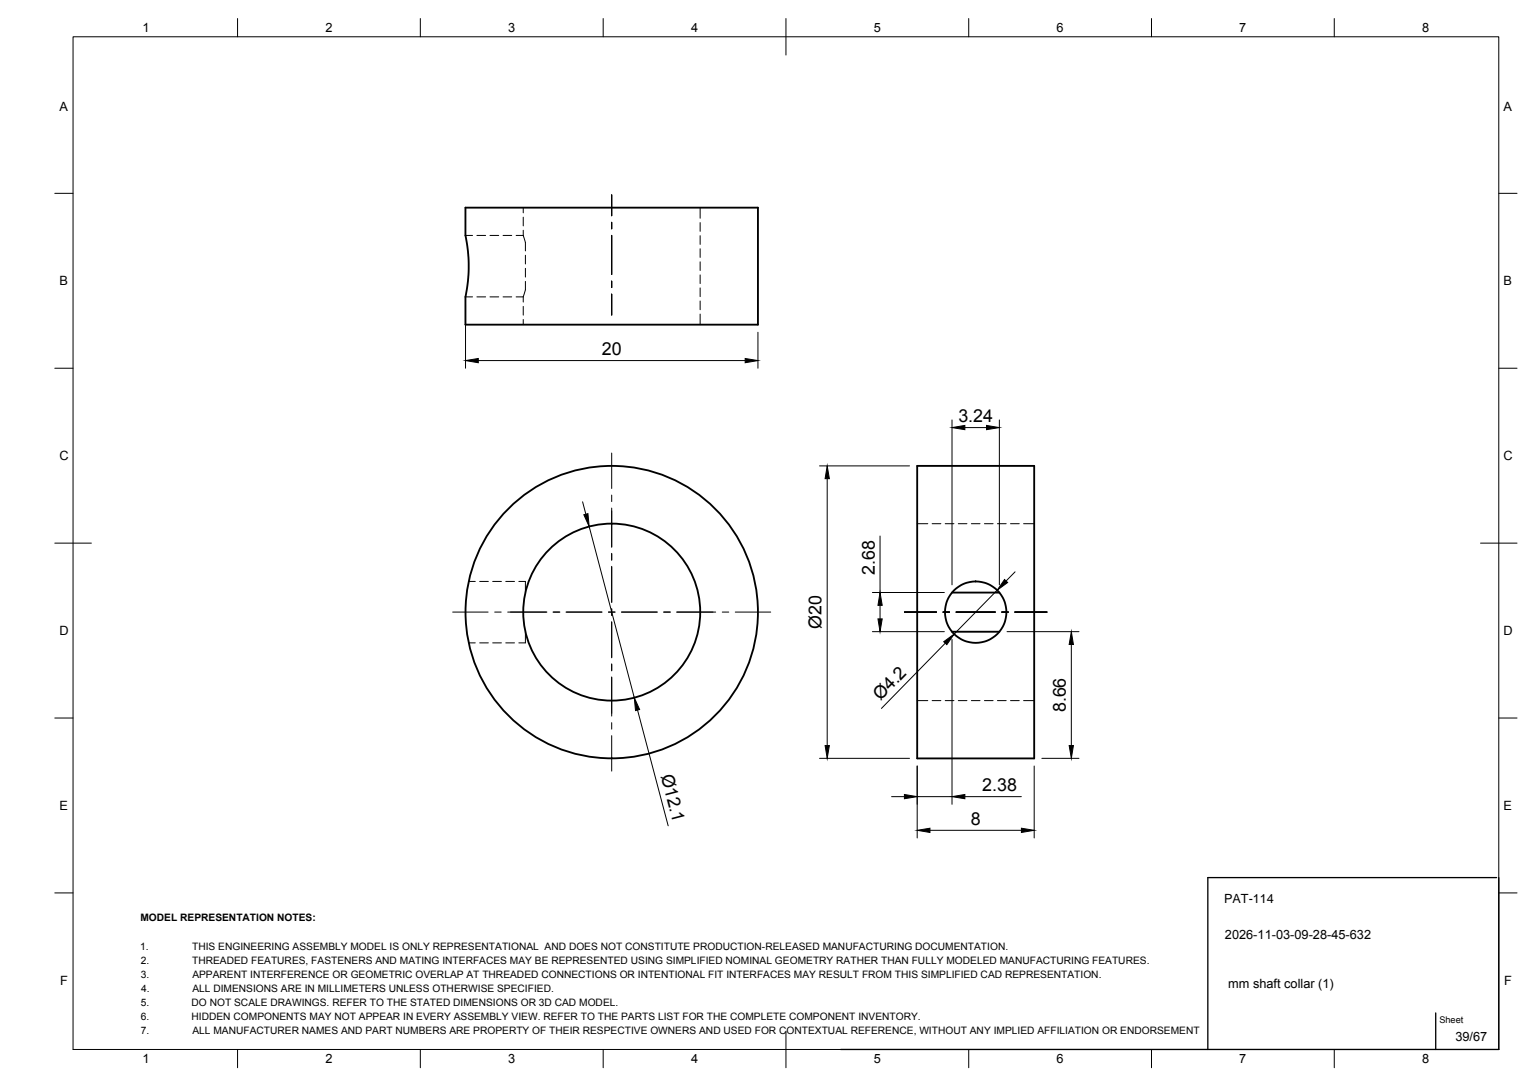
ISO-10303-21;
HEADER;
/* Generated by software containing ST-Developer
 * from STEP Tools, Inc. (www.steptools.com) 
 */

FILE_DESCRIPTION(
/* description */ ('Two-stage gear reducer in split housing'),
/* implementation_level */ '2;1');

FILE_NAME(
/* name */ 'mm shaft collar (1).step',
/* time_stamp */ '2026-10-28T03:22:31-07:00',
/* author */ (''),
/* organization */ (''),
/* preprocessor_version */ 'ST-DEVELOPER v20.2',
/* originating_system */ 'Autodesk Translation Framework v15.17.0.0',
/* authorisation */ '');

FILE_SCHEMA (('AUTOMOTIVE_DESIGN { 1 0 10303 214 3 1 1 }'));
ENDSEC;

DATA;
#10=MECHANICAL_DESIGN_GEOMETRIC_PRESENTATION_REPRESENTATION('',(#1279),#73366);
#967=B_SPLINE_CURVE_WITH_KNOTS('',3,(#25552,#25553,#25554,#25555,#25556,
#25557,#25558,#25559,#25560,#25561),.UNSPECIFIED.,.F.,.F.,(4,2,2,2,4),(0.818088904349178,
0.878131747417166,0.957937926194037,1.03774410497091,1.0977869480389),
 .UNSPECIFIED.);
#968=B_SPLINE_CURVE_WITH_KNOTS('',3,(#25567,#25568,#25569,#25570,#25571,
#25572,#25573,#25574,#25575,#25576,#25577,#25578,#25579,#25580,#25581,#25582,
#25583,#25584),.UNSPECIFIED.,.F.,.F.,(4,2,2,2,2,2,2,2,4),(0.,0.0793616477694788,
0.158723295538958,0.238079516586307,0.317435737633657,0.396791958681006,
0.476148179728355,0.555509827497834,0.634871475267313),.UNSPECIFIED.);
#969=B_SPLINE_CURVE_WITH_KNOTS('',3,(#25585,#25586,#25587,#25588,#25589,
#25590,#25591,#25592,#25593,#25594,#25595,#25596,#25597,#25598,#25599,#25600,
#25601,#25602),.UNSPECIFIED.,.F.,.F.,(4,2,2,2,2,2,2,2,4),(0.634871475267313,
0.714233123036792,0.79359477080627,0.87295099185362,0.95230721290097,1.03166343394832,
1.11101965499567,1.19038130276515,1.26974295053463),.UNSPECIFIED.);
#970=B_SPLINE_CURVE_WITH_KNOTS('',3,(#25605,#25606,#25607,#25608,#25609,
#25610,#25611,#25612,#25613,#25614),.UNSPECIFIED.,.F.,.F.,(4,2,2,2,4),(0.179463620219821,
0.239506463287808,0.319312642064679,0.39911882084155,0.459161663909537),
 .UNSPECIFIED.);
#1152=SHAPE_REPRESENTATION_RELATIONSHIP('SRR','None',#73642,#1208);
#1208=ADVANCED_BREP_SHAPE_REPRESENTATION('',(#1348),#73338);
#1279=STYLED_ITEM('',(#73988),#1348);
#1348=MANIFOLD_SOLID_BREP('Body1',#16169);
#1543=FACE_BOUND('',#3517,.T.);
#1544=FACE_BOUND('',#3519,.T.);
#1545=FACE_BOUND('',#3521,.T.);
#1546=FACE_BOUND('',#3523,.T.);
#1810=PLANE('',#17794);
#1811=PLANE('',#17799);
#1812=PLANE('',#17806);
#1813=PLANE('',#17807);
#2431=FACE_OUTER_BOUND('',#3513,.T.);
#2432=FACE_OUTER_BOUND('',#3514,.T.);
#2433=FACE_OUTER_BOUND('',#3515,.T.);
#2434=FACE_OUTER_BOUND('',#3516,.T.);
#2435=FACE_OUTER_BOUND('',#3518,.T.);
#2436=FACE_OUTER_BOUND('',#3520,.T.);
#2437=FACE_OUTER_BOUND('',#3522,.T.);
#3513=EDGE_LOOP('',(#12351,#12352));
#3514=EDGE_LOOP('',(#12353,#12354,#12355,#12356,#12357,#12358,#12359,#12360,
#12361));
#3515=EDGE_LOOP('',(#12362,#12363,#12364));
#3516=EDGE_LOOP('',(#12365,#12366,#12367,#12368));
#3517=EDGE_LOOP('',(#12369,#12370,#12371,#12372));
#3518=EDGE_LOOP('',(#12373,#12374,#12375,#12376));
#3519=EDGE_LOOP('',(#12377,#12378));
#3520=EDGE_LOOP('',(#12379));
#3521=EDGE_LOOP('',(#12380));
#3522=EDGE_LOOP('',(#12381));
#3523=EDGE_LOOP('',(#12382));
#4495=LINE('',#25548,#5519);
#4496=LINE('',#25565,#5520);
#4497=LINE('',#25616,#5521);
#4498=LINE('',#25621,#5522);
#4499=LINE('',#25627,#5523);
#5519=VECTOR('',#20863,1.);
#5520=VECTOR('',#20870,0.21);
#5521=VECTOR('',#20875,1.);
#5522=VECTOR('',#20880,0.605);
#5523=VECTOR('',#20887,1.);
#6551=CIRCLE('',#17795,0.21);
#6552=CIRCLE('',#17797,0.21);
#6553=CIRCLE('',#17798,0.21);
#6554=CIRCLE('',#17801,0.605);
#6555=CIRCLE('',#17802,0.605);
#6556=CIRCLE('',#17804,1.);
#6557=CIRCLE('',#17805,1.);
#7454=VERTEX_POINT('',#25546);
#7455=VERTEX_POINT('',#25547);
#7456=VERTEX_POINT('',#25551);
#7457=VERTEX_POINT('',#25562);
#7458=VERTEX_POINT('',#25564);
#7459=VERTEX_POINT('',#25566);
#7460=VERTEX_POINT('',#25603);
#7461=VERTEX_POINT('',#25618);
#7462=VERTEX_POINT('',#25620);
#7463=VERTEX_POINT('',#25624);
#7464=VERTEX_POINT('',#25626);
#9229=EDGE_CURVE('',#7454,#7455,#4495,.T.);
#9230=EDGE_CURVE('',#7454,#7455,#6551,.T.);
#9231=EDGE_CURVE('',#7456,#7454,#967,.T.);
#9232=EDGE_CURVE('',#7457,#7456,#6552,.T.);
#9233=EDGE_CURVE('',#7457,#7458,#4496,.T.);
#9234=EDGE_CURVE('',#7459,#7458,#968,.T.);
#9235=EDGE_CURVE('',#7458,#7459,#969,.T.);
#9236=EDGE_CURVE('',#7460,#7457,#6553,.T.);
#9237=EDGE_CURVE('',#7455,#7460,#970,.T.);
#9238=EDGE_CURVE('',#7460,#7456,#4497,.T.);
#9239=EDGE_CURVE('',#7461,#7461,#6554,.T.);
#9240=EDGE_CURVE('',#7461,#7462,#4498,.T.);
#9241=EDGE_CURVE('',#7462,#7462,#6555,.T.);
#9242=EDGE_CURVE('',#7463,#7463,#6556,.T.);
#9243=EDGE_CURVE('',#7463,#7464,#4499,.T.);
#9244=EDGE_CURVE('',#7464,#7464,#6557,.T.);
#12351=ORIENTED_EDGE('',*,*,#9229,.F.);
#12352=ORIENTED_EDGE('',*,*,#9230,.T.);
#12353=ORIENTED_EDGE('',*,*,#9231,.F.);
#12354=ORIENTED_EDGE('',*,*,#9232,.F.);
#12355=ORIENTED_EDGE('',*,*,#9233,.T.);
#12356=ORIENTED_EDGE('',*,*,#9234,.F.);
#12357=ORIENTED_EDGE('',*,*,#9235,.F.);
#12358=ORIENTED_EDGE('',*,*,#9233,.F.);
#12359=ORIENTED_EDGE('',*,*,#9236,.F.);
#12360=ORIENTED_EDGE('',*,*,#9237,.F.);
#12361=ORIENTED_EDGE('',*,*,#9230,.F.);
#12362=ORIENTED_EDGE('',*,*,#9238,.F.);
#12363=ORIENTED_EDGE('',*,*,#9236,.T.);
#12364=ORIENTED_EDGE('',*,*,#9232,.T.);
#12365=ORIENTED_EDGE('',*,*,#9239,.F.);
#12366=ORIENTED_EDGE('',*,*,#9240,.T.);
#12367=ORIENTED_EDGE('',*,*,#9241,.T.);
#12368=ORIENTED_EDGE('',*,*,#9240,.F.);
#12369=ORIENTED_EDGE('',*,*,#9237,.T.);
#12370=ORIENTED_EDGE('',*,*,#9238,.T.);
#12371=ORIENTED_EDGE('',*,*,#9231,.T.);
#12372=ORIENTED_EDGE('',*,*,#9229,.T.);
#12373=ORIENTED_EDGE('',*,*,#9242,.F.);
#12374=ORIENTED_EDGE('',*,*,#9243,.T.);
#12375=ORIENTED_EDGE('',*,*,#9244,.T.);
#12376=ORIENTED_EDGE('',*,*,#9243,.F.);
#12377=ORIENTED_EDGE('',*,*,#9234,.T.);
#12378=ORIENTED_EDGE('',*,*,#9235,.T.);
#12379=ORIENTED_EDGE('',*,*,#9242,.T.);
#12380=ORIENTED_EDGE('',*,*,#9239,.T.);
#12381=ORIENTED_EDGE('',*,*,#9244,.F.);
#12382=ORIENTED_EDGE('',*,*,#9241,.F.);
#15079=CYLINDRICAL_SURFACE('',#17796,0.21);
#15080=CYLINDRICAL_SURFACE('',#17800,0.605);
#15081=CYLINDRICAL_SURFACE('',#17803,1.);
#15638=ADVANCED_FACE('',(#2431),#1810,.T.);
#15639=ADVANCED_FACE('',(#2432),#15079,.F.);
#15640=ADVANCED_FACE('',(#2433),#1811,.T.);
#15641=ADVANCED_FACE('',(#2434,#1543),#15080,.F.);
#15642=ADVANCED_FACE('',(#2435,#1544),#15081,.T.);
#15643=ADVANCED_FACE('',(#2436,#1545),#1812,.T.);
#15644=ADVANCED_FACE('',(#2437,#1546),#1813,.F.);
#16169=CLOSED_SHELL('',(#15638,#15639,#15640,#15641,#15642,#15643,#15644));
#17793=AXIS2_PLACEMENT_3D('',#25544,#20859,#20860);
#17794=AXIS2_PLACEMENT_3D('',#25545,#20861,#20862);
#17795=AXIS2_PLACEMENT_3D('',#25549,#20864,#20865);
#17796=AXIS2_PLACEMENT_3D('',#25550,#20866,#20867);
#17797=AXIS2_PLACEMENT_3D('',#25563,#20868,#20869);
#17798=AXIS2_PLACEMENT_3D('',#25604,#20871,#20872);
#17799=AXIS2_PLACEMENT_3D('',#25615,#20873,#20874);
#17800=AXIS2_PLACEMENT_3D('',#25617,#20876,#20877);
#17801=AXIS2_PLACEMENT_3D('',#25619,#20878,#20879);
#17802=AXIS2_PLACEMENT_3D('',#25622,#20881,#20882);
#17803=AXIS2_PLACEMENT_3D('',#25623,#20883,#20884);
#17804=AXIS2_PLACEMENT_3D('',#25625,#20885,#20886);
#17805=AXIS2_PLACEMENT_3D('',#25628,#20888,#20889);
#17806=AXIS2_PLACEMENT_3D('',#25629,#20890,#20891);
#17807=AXIS2_PLACEMENT_3D('',#25630,#20892,#20893);
#20859=DIRECTION('axis',(0.,0.,1.));
#20860=DIRECTION('refdir',(1.,0.,0.));
#20861=DIRECTION('center_axis',(0.,0.,1.));
#20862=DIRECTION('ref_axis',(1.,0.,0.));
#20863=DIRECTION('',(0.,1.,0.));
#20864=DIRECTION('center_axis',(0.,0.,1.));
#20865=DIRECTION('ref_axis',(1.,0.,0.));
#20866=DIRECTION('center_axis',(0.,0.,1.));
#20867=DIRECTION('ref_axis',(1.,0.,0.));
#20868=DIRECTION('center_axis',(0.,0.,1.));
#20869=DIRECTION('ref_axis',(1.,0.,0.));
#20870=DIRECTION('',(0.,0.,1.));
#20871=DIRECTION('center_axis',(0.,0.,1.));
#20872=DIRECTION('ref_axis',(1.,0.,0.));
#20873=DIRECTION('center_axis',(0.,0.,1.));
#20874=DIRECTION('ref_axis',(1.,0.,0.));
#20875=DIRECTION('',(0.,-1.,0.));
#20876=DIRECTION('center_axis',(0.,1.,0.));
#20877=DIRECTION('ref_axis',(1.,0.,0.));
#20878=DIRECTION('center_axis',(0.,-1.,0.));
#20879=DIRECTION('ref_axis',(1.,0.,0.));
#20880=DIRECTION('',(0.,-1.,0.));
#20881=DIRECTION('center_axis',(0.,-1.,0.));
#20882=DIRECTION('ref_axis',(1.,0.,0.));
#20883=DIRECTION('center_axis',(0.,1.,0.));
#20884=DIRECTION('ref_axis',(1.,0.,0.));
#20885=DIRECTION('center_axis',(0.,1.,0.));
#20886=DIRECTION('ref_axis',(1.,0.,0.));
#20887=DIRECTION('',(0.,-1.,0.));
#20888=DIRECTION('center_axis',(0.,1.,0.));
#20889=DIRECTION('ref_axis',(1.,0.,0.));
#20890=DIRECTION('center_axis',(0.,1.,0.));
#20891=DIRECTION('ref_axis',(1.,0.,0.));
#20892=DIRECTION('center_axis',(0.,1.,0.));
#20893=DIRECTION('ref_axis',(1.,0.,0.));
#25544=CARTESIAN_POINT('',(0.,0.,0.));
#25545=CARTESIAN_POINT('Origin',(0.,8.2,10.59));
#25546=CARTESIAN_POINT('',(0.133884278389952,8.03821310312636,10.59));
#25547=CARTESIAN_POINT('',(0.133884278389952,8.36178689687364,10.59));
#25548=CARTESIAN_POINT('',(0.133884278389952,7.8,10.59));
#25549=CARTESIAN_POINT('Origin',(0.,8.2,10.59));
#25550=CARTESIAN_POINT('Origin',(0.,8.2,10.59));
#25551=CARTESIAN_POINT('',(-0.133884278389952,8.03821310312636,10.59));
#25552=CARTESIAN_POINT('Ctrl Pts',(-0.133884278389952,8.03821310312636,
10.59));
#25553=CARTESIAN_POINT('Ctrl Pts',(-0.118254395260798,8.02527883178237,
10.5935467722442));
#25554=CARTESIAN_POINT('Ctrl Pts',(-0.100109787682297,8.01420068341256,
10.5969822478996));
#25555=CARTESIAN_POINT('Ctrl Pts',(-0.0548298721325187,7.99536143894557,
10.6030741628997));
#25556=CARTESIAN_POINT('Ctrl Pts',(-0.0266020595922903,7.99,10.605));
#25557=CARTESIAN_POINT('Ctrl Pts',(0.0266020595922902,7.99,10.605));
#25558=CARTESIAN_POINT('Ctrl Pts',(0.0548298721325187,7.99536143894557,
10.6030741628997));
#25559=CARTESIAN_POINT('Ctrl Pts',(0.100109787682297,8.01420068341256,10.5969822478996));
#25560=CARTESIAN_POINT('Ctrl Pts',(0.118254395260798,8.02527883178237,10.5935467722442));
#25561=CARTESIAN_POINT('Ctrl Pts',(0.133884278389952,8.03821310312636,10.59));
#25562=CARTESIAN_POINT('',(-0.21,8.2,10.59));
#25563=CARTESIAN_POINT('Origin',(0.,8.2,10.59));
#25564=CARTESIAN_POINT('',(-0.21,8.2,10.9777013859047));
#25565=CARTESIAN_POINT('',(-0.21,8.2,10.59));
#25566=CARTESIAN_POINT('',(0.21,8.2,10.9777013859047));
#25567=CARTESIAN_POINT('Ctrl Pts',(0.21,8.2,10.9777013859047));
#25568=CARTESIAN_POINT('Ctrl Pts',(0.21,8.17354611741017,10.9777013859047));
#25569=CARTESIAN_POINT('Ctrl Pts',(0.204697017125528,8.14538474169131,10.9788864661322));
#25570=CARTESIAN_POINT('Ctrl Pts',(0.18324175151553,8.09366957869826,10.9831286999115));
#25571=CARTESIAN_POINT('Ctrl Pts',(0.167093586802907,8.07010873870455,10.9861204479665));
#25572=CARTESIAN_POINT('Ctrl Pts',(0.129892533236543,8.03290768513819,10.9917064515638));
#25573=CARTESIAN_POINT('Ctrl Pts',(0.106331154992713,8.01675852489431,10.994669144466));
#25574=CARTESIAN_POINT('Ctrl Pts',(0.0546141143983529,7.99530253627557,
10.9988444923724));
#25575=CARTESIAN_POINT('Ctrl Pts',(0.0264520736824498,7.99,11.));
#25576=CARTESIAN_POINT('Ctrl Pts',(-0.0264520736824498,7.99,11.));
#25577=CARTESIAN_POINT('Ctrl Pts',(-0.0546141143983529,7.99530253627557,
10.9988444923724));
#25578=CARTESIAN_POINT('Ctrl Pts',(-0.106331154992713,8.01675852489431,
10.994669144466));
#25579=CARTESIAN_POINT('Ctrl Pts',(-0.129892533236543,8.03290768513819,
10.9917064515638));
#25580=CARTESIAN_POINT('Ctrl Pts',(-0.167093586802907,8.07010873870455,
10.9861204479665));
#25581=CARTESIAN_POINT('Ctrl Pts',(-0.18324175151553,8.09366957869826,10.9831286999115));
#25582=CARTESIAN_POINT('Ctrl Pts',(-0.204697017125528,8.14538474169131,
10.9788864661322));
#25583=CARTESIAN_POINT('Ctrl Pts',(-0.21,8.17354611741017,10.9777013859047));
#25584=CARTESIAN_POINT('Ctrl Pts',(-0.21,8.2,10.9777013859047));
#25585=CARTESIAN_POINT('Ctrl Pts',(-0.21,8.2,10.9777013859047));
#25586=CARTESIAN_POINT('Ctrl Pts',(-0.21,8.22645388258983,10.9777013859047));
#25587=CARTESIAN_POINT('Ctrl Pts',(-0.204697017125528,8.25461525830868,
10.9788864661322));
#25588=CARTESIAN_POINT('Ctrl Pts',(-0.18324175151553,8.30633042130174,10.9831286999115));
#25589=CARTESIAN_POINT('Ctrl Pts',(-0.167093586802906,8.32989126129544,
10.9861204479665));
#25590=CARTESIAN_POINT('Ctrl Pts',(-0.129892533236543,8.36709231486181,
10.9917064515638));
#25591=CARTESIAN_POINT('Ctrl Pts',(-0.106331154992713,8.38324147510569,
10.994669144466));
#25592=CARTESIAN_POINT('Ctrl Pts',(-0.0546141143983529,8.40469746372443,
10.9988444923724));
#25593=CARTESIAN_POINT('Ctrl Pts',(-0.0264520736824499,8.41,11.));
#25594=CARTESIAN_POINT('Ctrl Pts',(0.0264520736824498,8.41,11.));
#25595=CARTESIAN_POINT('Ctrl Pts',(0.0546141143983528,8.40469746372443,
10.9988444923724));
#25596=CARTESIAN_POINT('Ctrl Pts',(0.106331154992713,8.38324147510569,10.994669144466));
#25597=CARTESIAN_POINT('Ctrl Pts',(0.129892533236543,8.36709231486181,10.9917064515638));
#25598=CARTESIAN_POINT('Ctrl Pts',(0.167093586802906,8.32989126129544,10.9861204479665));
#25599=CARTESIAN_POINT('Ctrl Pts',(0.18324175151553,8.30633042130174,10.9831286999115));
#25600=CARTESIAN_POINT('Ctrl Pts',(0.204697017125528,8.25461525830868,10.9788864661322));
#25601=CARTESIAN_POINT('Ctrl Pts',(0.21,8.22645388258983,10.9777013859047));
#25602=CARTESIAN_POINT('Ctrl Pts',(0.21,8.2,10.9777013859047));
#25603=CARTESIAN_POINT('',(-0.133884278389952,8.36178689687364,10.59));
#25604=CARTESIAN_POINT('Origin',(0.,8.2,10.59));
#25605=CARTESIAN_POINT('Ctrl Pts',(0.133884278389952,8.36178689687364,10.59));
#25606=CARTESIAN_POINT('Ctrl Pts',(0.1182543952608,8.37472116821763,10.5935467722442));
#25607=CARTESIAN_POINT('Ctrl Pts',(0.100109787682296,8.38579931658744,10.5969822478996));
#25608=CARTESIAN_POINT('Ctrl Pts',(0.0548298721325181,8.40463856105443,
10.6030741628997));
#25609=CARTESIAN_POINT('Ctrl Pts',(0.0266020595922904,8.41,10.605));
#25610=CARTESIAN_POINT('Ctrl Pts',(-0.0266020595922903,8.41,10.605));
#25611=CARTESIAN_POINT('Ctrl Pts',(-0.0548298721325181,8.40463856105443,
10.6030741628997));
#25612=CARTESIAN_POINT('Ctrl Pts',(-0.100109787682296,8.38579931658744,
10.5969822478996));
#25613=CARTESIAN_POINT('Ctrl Pts',(-0.118254395260799,8.37472116821763,
10.5935467722442));
#25614=CARTESIAN_POINT('Ctrl Pts',(-0.133884278389951,8.36178689687364,
10.59));
#25615=CARTESIAN_POINT('Origin',(0.,8.2,10.59));
#25616=CARTESIAN_POINT('',(-0.133884278389952,7.8,10.59));
#25617=CARTESIAN_POINT('Origin',(0.,7.8,10.));
#25618=CARTESIAN_POINT('',(-0.605,8.6,10.));
#25619=CARTESIAN_POINT('Origin',(0.,8.6,10.));
#25620=CARTESIAN_POINT('',(-0.605,7.8,10.));
#25621=CARTESIAN_POINT('',(-0.605,7.8,10.));
#25622=CARTESIAN_POINT('Origin',(0.,7.8,10.));
#25623=CARTESIAN_POINT('Origin',(0.,7.8,10.));
#25624=CARTESIAN_POINT('',(-1.,8.6,10.));
#25625=CARTESIAN_POINT('Origin',(0.,8.6,10.));
#25626=CARTESIAN_POINT('',(-1.,7.8,10.));
#25627=CARTESIAN_POINT('',(-1.,7.8,10.));
#25628=CARTESIAN_POINT('Origin',(0.,7.8,10.));
#25629=CARTESIAN_POINT('Origin',(0.,8.6,10.));
#25630=CARTESIAN_POINT('Origin',(0.,7.8,10.));
#73274=UNCERTAINTY_MEASURE_WITH_UNIT(LENGTH_MEASURE(0.001),#73367,
'DISTANCE_ACCURACY_VALUE',
'Maximum model space distance between geometric entities at asserted c
onnectivities');
#73302=UNCERTAINTY_MEASURE_WITH_UNIT(LENGTH_MEASURE(0.001),#73367,
'DISTANCE_ACCURACY_VALUE',
'Maximum model space distance between geometric entities at asserted c
onnectivities');
#73338=(
GEOMETRIC_REPRESENTATION_CONTEXT(3)
GLOBAL_UNCERTAINTY_ASSIGNED_CONTEXT((#73274))
GLOBAL_UNIT_ASSIGNED_CONTEXT((#73367,#73369,#73370))
REPRESENTATION_CONTEXT('','3D')
);
#73366=(
GEOMETRIC_REPRESENTATION_CONTEXT(3)
GLOBAL_UNCERTAINTY_ASSIGNED_CONTEXT((#73302))
GLOBAL_UNIT_ASSIGNED_CONTEXT((#73367,#73369,#73370))
REPRESENTATION_CONTEXT('','3D')
);
#73367=(
LENGTH_UNIT()
NAMED_UNIT(*)
SI_UNIT(.CENTI.,.METRE.)
);
#73369=(
NAMED_UNIT(*)
PLANE_ANGLE_UNIT()
SI_UNIT($,.RADIAN.)
);
#73370=(
NAMED_UNIT(*)
SI_UNIT($,.STERADIAN.)
SOLID_ANGLE_UNIT()
);
#73406=SHAPE_DEFINITION_REPRESENTATION(#73539,#73642);
#73539=PRODUCT_DEFINITION_SHAPE('',$,#73706);
#73642=SHAPE_REPRESENTATION('',(#17793),#73338);
#73670=PRODUCT_DEFINITION_CONTEXT('part definition',#73861,'design');
#73706=PRODUCT_DEFINITION('mm shaft collar (1)','mm shaft collar (1)',#73769,
#73670);
#73769=PRODUCT_DEFINITION_FORMATION('',$,#73898);
#73861=APPLICATION_CONTEXT(
'Core Data for Automotive Mechanical Design Process');
#73862=PRODUCT_CONTEXT('part definition',#73861,'mechanical');
#73898=PRODUCT('mm shaft collar (1)','mm shaft collar (1)',
'mm shaft collar (1)',(#73862));
#73982=COLOUR_RGB('Grey',0.48,0.52,0.57);
#73983=FILL_AREA_STYLE_COLOUR('',#73982);
#73984=FILL_AREA_STYLE('',(#73983));
#73985=SURFACE_STYLE_FILL_AREA(#73984);
#73986=SURFACE_SIDE_STYLE('',(#73985));
#73987=SURFACE_STYLE_USAGE(.BOTH.,#73986);
#73988=PRESENTATION_STYLE_ASSIGNMENT((#73987));
ENDSEC;
END-ISO-10303-21;
